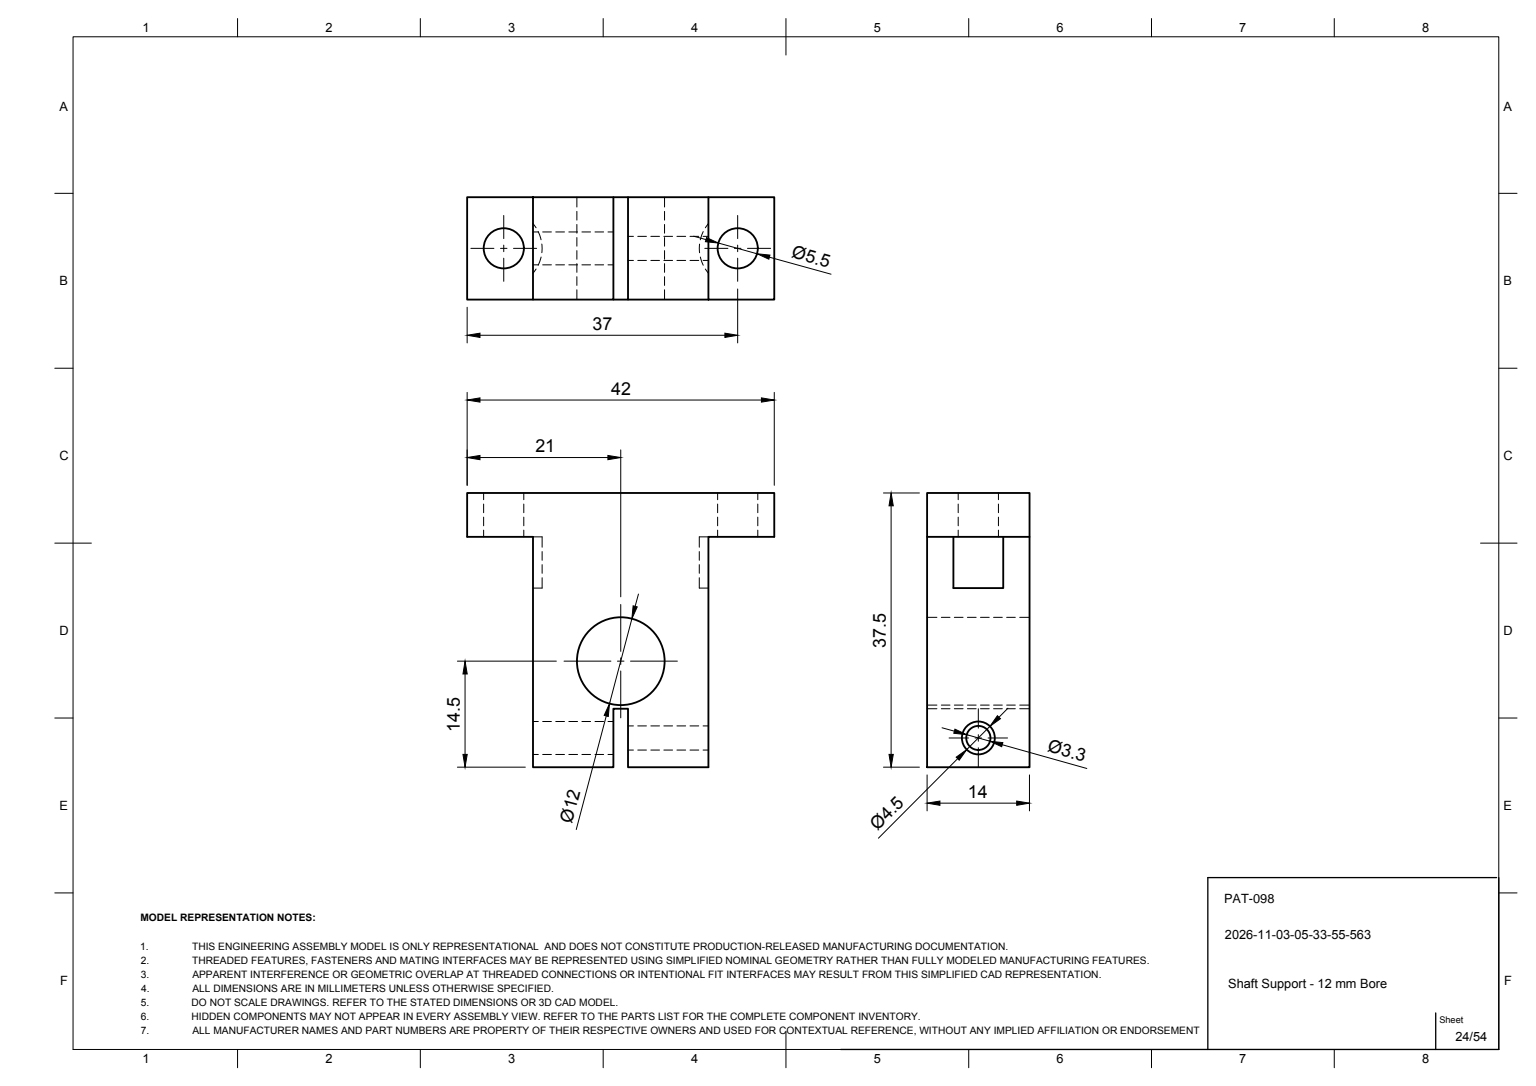
ISO-10303-21;
HEADER;
/* Generated by software containing ST-Developer
 * from STEP Tools, Inc. (www.steptools.com) 
 */

FILE_DESCRIPTION(
/* description */ ('Spring compression tester'),
/* implementation_level */ '2;1');

FILE_NAME(
/* name */ 'Shaft Support - 12 mm Bore.step',
/* time_stamp */ '2026-10-28T03:24:11-07:00',
/* author */ (''),
/* organization */ (''),
/* preprocessor_version */ 'ST-DEVELOPER v20.2',
/* originating_system */ 'Autodesk Translation Framework v15.17.0.0',
/* authorisation */ '');

FILE_SCHEMA (('AUTOMOTIVE_DESIGN { 1 0 10303 214 3 1 1 }'));
ENDSEC;

DATA;
#10=MECHANICAL_DESIGN_GEOMETRIC_PRESENTATION_REPRESENTATION('',(#1125),#43521);
#1005=SHAPE_REPRESENTATION_RELATIONSHIP('SRR','None',#43817,#1065);
#1065=ADVANCED_BREP_SHAPE_REPRESENTATION('',(#1200),#43477);
#1125=STYLED_ITEM('',(#44202),#1200);
#1200=MANIFOLD_SOLID_BREP('Body1',#18562);
#1439=FACE_BOUND('',#3801,.T.);
#1440=FACE_BOUND('',#3803,.T.);
#1441=FACE_BOUND('',#3805,.T.);
#1442=FACE_BOUND('',#3812,.T.);
#1443=FACE_BOUND('',#3815,.T.);
#1444=FACE_BOUND('',#3816,.T.);
#1445=FACE_BOUND('',#3819,.T.);
#1446=FACE_BOUND('',#3822,.T.);
#1447=FACE_BOUND('',#3825,.T.);
#1448=FACE_BOUND('',#3828,.T.);
#1861=PLANE('',#19931);
#1862=PLANE('',#19938);
#1863=PLANE('',#19939);
#1864=PLANE('',#19941);
#1865=PLANE('',#19943);
#1866=PLANE('',#19957);
#1867=PLANE('',#19958);
#1868=PLANE('',#19959);
#1869=PLANE('',#19960);
#1870=PLANE('',#19961);
#1871=PLANE('',#19962);
#1872=PLANE('',#19963);
#1873=PLANE('',#19964);
#1874=PLANE('',#19965);
#1875=PLANE('',#19966);
#1876=PLANE('',#19967);
#2557=FACE_OUTER_BOUND('',#3796,.T.);
#2558=FACE_OUTER_BOUND('',#3797,.T.);
#2559=FACE_OUTER_BOUND('',#3798,.T.);
#2560=FACE_OUTER_BOUND('',#3799,.T.);
#2561=FACE_OUTER_BOUND('',#3800,.T.);
#2562=FACE_OUTER_BOUND('',#3802,.T.);
#2563=FACE_OUTER_BOUND('',#3804,.T.);
#2564=FACE_OUTER_BOUND('',#3806,.T.);
#2565=FACE_OUTER_BOUND('',#3807,.T.);
#2566=FACE_OUTER_BOUND('',#3808,.T.);
#2567=FACE_OUTER_BOUND('',#3809,.T.);
#2568=FACE_OUTER_BOUND('',#3810,.T.);
#2569=FACE_OUTER_BOUND('',#3811,.T.);
#2570=FACE_OUTER_BOUND('',#3813,.T.);
#2571=FACE_OUTER_BOUND('',#3814,.T.);
#2572=FACE_OUTER_BOUND('',#3817,.T.);
#2573=FACE_OUTER_BOUND('',#3818,.T.);
#2574=FACE_OUTER_BOUND('',#3820,.T.);
#2575=FACE_OUTER_BOUND('',#3821,.T.);
#2576=FACE_OUTER_BOUND('',#3823,.T.);
#2577=FACE_OUTER_BOUND('',#3824,.T.);
#2578=FACE_OUTER_BOUND('',#3826,.T.);
#2579=FACE_OUTER_BOUND('',#3827,.T.);
#3796=EDGE_LOOP('',(#13935,#13936));
#3797=EDGE_LOOP('',(#13937,#13938,#13939,#13940));
#3798=EDGE_LOOP('',(#13941,#13942,#13943,#13944));
#3799=EDGE_LOOP('',(#13945,#13946));
#3800=EDGE_LOOP('',(#13947,#13948,#13949,#13950,#13951,#13952));
#3801=EDGE_LOOP('',(#13953));
#3802=EDGE_LOOP('',(#13954,#13955,#13956,#13957,#13958,#13959,#13960,#13961));
#3803=EDGE_LOOP('',(#13962));
#3804=EDGE_LOOP('',(#13963,#13964,#13965,#13966,#13967,#13968));
#3805=EDGE_LOOP('',(#13969));
#3806=EDGE_LOOP('',(#13970,#13971,#13972,#13973));
#3807=EDGE_LOOP('',(#13974,#13975,#13976,#13977));
#3808=EDGE_LOOP('',(#13978,#13979,#13980,#13981));
#3809=EDGE_LOOP('',(#13982,#13983,#13984,#13985));
#3810=EDGE_LOOP('',(#13986,#13987,#13988,#13989));
#3811=EDGE_LOOP('',(#13990,#13991,#13992,#13993,#13994,#13995,#13996,#13997,
#13998,#13999,#14000,#14001));
#3812=EDGE_LOOP('',(#14002));
#3813=EDGE_LOOP('',(#14003,#14004,#14005,#14006));
#3814=EDGE_LOOP('',(#14007,#14008,#14009,#14010));
#3815=EDGE_LOOP('',(#14011));
#3816=EDGE_LOOP('',(#14012));
#3817=EDGE_LOOP('',(#14013,#14014,#14015,#14016));
#3818=EDGE_LOOP('',(#14017,#14018,#14019,#14020,#14021,#14022,#14023,#14024));
#3819=EDGE_LOOP('',(#14025));
#3820=EDGE_LOOP('',(#14026,#14027,#14028,#14029));
#3821=EDGE_LOOP('',(#14030,#14031,#14032,#14033));
#3822=EDGE_LOOP('',(#14034));
#3823=EDGE_LOOP('',(#14035,#14036,#14037,#14038));
#3824=EDGE_LOOP('',(#14039,#14040,#14041,#14042));
#3825=EDGE_LOOP('',(#14043));
#3826=EDGE_LOOP('',(#14044,#14045,#14046,#14047));
#3827=EDGE_LOOP('',(#14048,#14049,#14050,#14051,#14052,#14053,#14054,#14055,
#14056,#14057,#14058,#14059));
#3828=EDGE_LOOP('',(#14060));
#5229=LINE('',#28297,#6661);
#5230=LINE('',#28301,#6662);
#5231=LINE('',#28304,#6663);
#5232=LINE('',#28308,#6664);
#5233=LINE('',#28312,#6665);
#5234=LINE('',#28315,#6666);
#5235=LINE('',#28318,#6667);
#5236=LINE('',#28320,#6668);
#5237=LINE('',#28322,#6669);
#5238=LINE('',#28324,#6670);
#5239=LINE('',#28325,#6671);
#5240=LINE('',#28330,#6672);
#5241=LINE('',#28332,#6673);
#5242=LINE('',#28333,#6674);
#5243=LINE('',#28339,#6675);
#5244=LINE('',#28341,#6676);
#5245=LINE('',#28342,#6677);
#5246=LINE('',#28344,#6678);
#5247=LINE('',#28345,#6679);
#5248=LINE('',#28352,#6680);
#5249=LINE('',#28356,#6681);
#5250=LINE('',#28361,#6682);
#5251=LINE('',#28365,#6683);
#5252=LINE('',#28370,#6684);
#5253=LINE('',#28374,#6685);
#5254=LINE('',#28376,#6686);
#5255=LINE('',#28377,#6687);
#5256=LINE('',#28379,#6688);
#5257=LINE('',#28381,#6689);
#5258=LINE('',#28383,#6690);
#5259=LINE('',#28385,#6691);
#5260=LINE('',#28387,#6692);
#5261=LINE('',#28388,#6693);
#5262=LINE('',#28391,#6694);
#5263=LINE('',#28392,#6695);
#5264=LINE('',#28395,#6696);
#5265=LINE('',#28396,#6697);
#5266=LINE('',#28398,#6698);
#5267=LINE('',#28401,#6699);
#5268=LINE('',#28402,#6700);
#5269=LINE('',#28405,#6701);
#5270=LINE('',#28406,#6702);
#5271=LINE('',#28409,#6703);
#5272=LINE('',#28410,#6704);
#5273=LINE('',#28413,#6705);
#5274=LINE('',#28414,#6706);
#5275=LINE('',#28417,#6707);
#5276=LINE('',#28418,#6708);
#5277=LINE('',#28420,#6709);
#6661=VECTOR('',#23115,1.);
#6662=VECTOR('',#23120,1.);
#6663=VECTOR('',#23123,1.);
#6664=VECTOR('',#23126,1.);
#6665=VECTOR('',#23129,1.);
#6666=VECTOR('',#23134,1.);
#6667=VECTOR('',#23137,1.);
#6668=VECTOR('',#23138,1.);
#6669=VECTOR('',#23139,1.);
#6670=VECTOR('',#23140,1.);
#6671=VECTOR('',#23141,1.);
#6672=VECTOR('',#23146,1.);
#6673=VECTOR('',#23147,1.);
#6674=VECTOR('',#23148,1.);
#6675=VECTOR('',#23153,1.);
#6676=VECTOR('',#23154,1.);
#6677=VECTOR('',#23155,1.);
#6678=VECTOR('',#23156,1.);
#6679=VECTOR('',#23157,1.);
#6680=VECTOR('',#23164,0.225);
#6681=VECTOR('',#23169,0.165);
#6682=VECTOR('',#23176,0.275);
#6683=VECTOR('',#23181,0.275);
#6684=VECTOR('',#23186,0.6);
#6685=VECTOR('',#23191,1.);
#6686=VECTOR('',#23192,1.);
#6687=VECTOR('',#23193,1.);
#6688=VECTOR('',#23194,1.);
#6689=VECTOR('',#23195,1.);
#6690=VECTOR('',#23196,1.);
#6691=VECTOR('',#23197,1.);
#6692=VECTOR('',#23198,1.);
#6693=VECTOR('',#23199,1.);
#6694=VECTOR('',#23202,1.);
#6695=VECTOR('',#23203,1.);
#6696=VECTOR('',#23206,1.);
#6697=VECTOR('',#23207,1.);
#6698=VECTOR('',#23210,1.);
#6699=VECTOR('',#23213,1.);
#6700=VECTOR('',#23214,1.);
#6701=VECTOR('',#23217,1.);
#6702=VECTOR('',#23218,1.);
#6703=VECTOR('',#23221,1.);
#6704=VECTOR('',#23222,1.);
#6705=VECTOR('',#23225,1.);
#6706=VECTOR('',#23226,1.);
#6707=VECTOR('',#23229,1.);
#6708=VECTOR('',#23230,1.);
#6709=VECTOR('',#23233,1.);
#7706=CIRCLE('',#19932,0.525);
#7707=CIRCLE('',#19934,0.525);
#7708=CIRCLE('',#19936,0.525);
#7709=CIRCLE('',#19937,0.525);
#7710=CIRCLE('',#19940,0.275);
#7711=CIRCLE('',#19942,0.165);
#7712=CIRCLE('',#19944,0.275);
#7713=CIRCLE('',#19946,0.225);
#7714=CIRCLE('',#19947,0.225);
#7715=CIRCLE('',#19949,0.165);
#7716=CIRCLE('',#19951,0.275);
#7717=CIRCLE('',#19953,0.275);
#7718=CIRCLE('',#19955,0.6);
#7719=CIRCLE('',#19956,0.6);
#8708=VERTEX_POINT('',#28295);
#8709=VERTEX_POINT('',#28296);
#8710=VERTEX_POINT('',#28300);
#8711=VERTEX_POINT('',#28302);
#8712=VERTEX_POINT('',#28306);
#8713=VERTEX_POINT('',#28307);
#8714=VERTEX_POINT('',#28309);
#8715=VERTEX_POINT('',#28311);
#8716=VERTEX_POINT('',#28317);
#8717=VERTEX_POINT('',#28319);
#8718=VERTEX_POINT('',#28321);
#8719=VERTEX_POINT('',#28323);
#8720=VERTEX_POINT('',#28326);
#8721=VERTEX_POINT('',#28329);
#8722=VERTEX_POINT('',#28331);
#8723=VERTEX_POINT('',#28334);
#8724=VERTEX_POINT('',#28337);
#8725=VERTEX_POINT('',#28338);
#8726=VERTEX_POINT('',#28340);
#8727=VERTEX_POINT('',#28343);
#8728=VERTEX_POINT('',#28346);
#8729=VERTEX_POINT('',#28349);
#8730=VERTEX_POINT('',#28351);
#8731=VERTEX_POINT('',#28355);
#8732=VERTEX_POINT('',#28359);
#8733=VERTEX_POINT('',#28363);
#8734=VERTEX_POINT('',#28367);
#8735=VERTEX_POINT('',#28369);
#8736=VERTEX_POINT('',#28373);
#8737=VERTEX_POINT('',#28375);
#8738=VERTEX_POINT('',#28378);
#8739=VERTEX_POINT('',#28380);
#8740=VERTEX_POINT('',#28382);
#8741=VERTEX_POINT('',#28384);
#8742=VERTEX_POINT('',#28386);
#8743=VERTEX_POINT('',#28390);
#8744=VERTEX_POINT('',#28394);
#8745=VERTEX_POINT('',#28400);
#8746=VERTEX_POINT('',#28404);
#8747=VERTEX_POINT('',#28408);
#8748=VERTEX_POINT('',#28412);
#8749=VERTEX_POINT('',#28416);
#10632=EDGE_CURVE('',#8708,#8709,#5229,.T.);
#10633=EDGE_CURVE('',#8709,#8708,#7706,.T.);
#10634=EDGE_CURVE('',#8710,#8708,#5230,.T.);
#10635=EDGE_CURVE('',#8711,#8710,#7707,.T.);
#10636=EDGE_CURVE('',#8709,#8711,#5231,.T.);
#10637=EDGE_CURVE('',#8712,#8713,#5232,.T.);
#10638=EDGE_CURVE('',#8712,#8714,#7708,.T.);
#10639=EDGE_CURVE('',#8715,#8714,#5233,.T.);
#10640=EDGE_CURVE('',#8713,#8715,#7709,.T.);
#10641=EDGE_CURVE('',#8714,#8712,#5234,.T.);
#10642=EDGE_CURVE('',#8710,#8716,#5235,.T.);
#10643=EDGE_CURVE('',#8717,#8716,#5236,.T.);
#10644=EDGE_CURVE('',#8717,#8718,#5237,.T.);
#10645=EDGE_CURVE('',#8719,#8718,#5238,.T.);
#10646=EDGE_CURVE('',#8719,#8711,#5239,.T.);
#10647=EDGE_CURVE('',#8720,#8720,#7710,.T.);
#10648=EDGE_CURVE('',#8721,#8719,#5240,.T.);
#10649=EDGE_CURVE('',#8721,#8722,#5241,.T.);
#10650=EDGE_CURVE('',#8716,#8722,#5242,.T.);
#10651=EDGE_CURVE('',#8723,#8723,#7711,.T.);
#10652=EDGE_CURVE('',#8724,#8725,#5243,.T.);
#10653=EDGE_CURVE('',#8726,#8725,#5244,.T.);
#10654=EDGE_CURVE('',#8713,#8726,#5245,.T.);
#10655=EDGE_CURVE('',#8727,#8715,#5246,.T.);
#10656=EDGE_CURVE('',#8724,#8727,#5247,.T.);
#10657=EDGE_CURVE('',#8728,#8728,#7712,.T.);
#10658=EDGE_CURVE('',#8729,#8729,#7713,.T.);
#10659=EDGE_CURVE('',#8729,#8730,#5248,.T.);
#10660=EDGE_CURVE('',#8730,#8730,#7714,.T.);
#10661=EDGE_CURVE('',#8723,#8731,#5249,.T.);
#10662=EDGE_CURVE('',#8731,#8731,#7715,.T.);
#10663=EDGE_CURVE('',#8732,#8732,#7716,.T.);
#10664=EDGE_CURVE('',#8732,#8720,#5250,.T.);
#10665=EDGE_CURVE('',#8733,#8733,#7717,.T.);
#10666=EDGE_CURVE('',#8733,#8728,#5251,.T.);
#10667=EDGE_CURVE('',#8734,#8734,#7718,.T.);
#10668=EDGE_CURVE('',#8734,#8735,#5252,.T.);
#10669=EDGE_CURVE('',#8735,#8735,#7719,.T.);
#10670=EDGE_CURVE('',#8718,#8736,#5253,.T.);
#10671=EDGE_CURVE('',#8736,#8737,#5254,.T.);
#10672=EDGE_CURVE('',#8737,#8724,#5255,.T.);
#10673=EDGE_CURVE('',#8727,#8738,#5256,.T.);
#10674=EDGE_CURVE('',#8738,#8739,#5257,.T.);
#10675=EDGE_CURVE('',#8739,#8740,#5258,.T.);
#10676=EDGE_CURVE('',#8740,#8741,#5259,.T.);
#10677=EDGE_CURVE('',#8741,#8742,#5260,.T.);
#10678=EDGE_CURVE('',#8742,#8721,#5261,.T.);
#10679=EDGE_CURVE('',#8743,#8717,#5262,.T.);
#10680=EDGE_CURVE('',#8736,#8743,#5263,.T.);
#10681=EDGE_CURVE('',#8744,#8743,#5264,.T.);
#10682=EDGE_CURVE('',#8737,#8744,#5265,.T.);
#10683=EDGE_CURVE('',#8725,#8744,#5266,.T.);
#10684=EDGE_CURVE('',#8745,#8726,#5267,.T.);
#10685=EDGE_CURVE('',#8738,#8745,#5268,.T.);
#10686=EDGE_CURVE('',#8746,#8745,#5269,.T.);
#10687=EDGE_CURVE('',#8739,#8746,#5270,.T.);
#10688=EDGE_CURVE('',#8747,#8746,#5271,.T.);
#10689=EDGE_CURVE('',#8740,#8747,#5272,.T.);
#10690=EDGE_CURVE('',#8748,#8747,#5273,.T.);
#10691=EDGE_CURVE('',#8741,#8748,#5274,.T.);
#10692=EDGE_CURVE('',#8749,#8748,#5275,.T.);
#10693=EDGE_CURVE('',#8742,#8749,#5276,.T.);
#10694=EDGE_CURVE('',#8722,#8749,#5277,.T.);
#13935=ORIENTED_EDGE('',*,*,#10632,.F.);
#13936=ORIENTED_EDGE('',*,*,#10633,.F.);
#13937=ORIENTED_EDGE('',*,*,#10634,.F.);
#13938=ORIENTED_EDGE('',*,*,#10635,.F.);
#13939=ORIENTED_EDGE('',*,*,#10636,.F.);
#13940=ORIENTED_EDGE('',*,*,#10633,.T.);
#13941=ORIENTED_EDGE('',*,*,#10637,.F.);
#13942=ORIENTED_EDGE('',*,*,#10638,.T.);
#13943=ORIENTED_EDGE('',*,*,#10639,.F.);
#13944=ORIENTED_EDGE('',*,*,#10640,.F.);
#13945=ORIENTED_EDGE('',*,*,#10641,.F.);
#13946=ORIENTED_EDGE('',*,*,#10638,.F.);
#13947=ORIENTED_EDGE('',*,*,#10642,.T.);
#13948=ORIENTED_EDGE('',*,*,#10643,.F.);
#13949=ORIENTED_EDGE('',*,*,#10644,.T.);
#13950=ORIENTED_EDGE('',*,*,#10645,.F.);
#13951=ORIENTED_EDGE('',*,*,#10646,.T.);
#13952=ORIENTED_EDGE('',*,*,#10635,.T.);
#13953=ORIENTED_EDGE('',*,*,#10647,.T.);
#13954=ORIENTED_EDGE('',*,*,#10634,.T.);
#13955=ORIENTED_EDGE('',*,*,#10632,.T.);
#13956=ORIENTED_EDGE('',*,*,#10636,.T.);
#13957=ORIENTED_EDGE('',*,*,#10646,.F.);
#13958=ORIENTED_EDGE('',*,*,#10648,.F.);
#13959=ORIENTED_EDGE('',*,*,#10649,.T.);
#13960=ORIENTED_EDGE('',*,*,#10650,.F.);
#13961=ORIENTED_EDGE('',*,*,#10642,.F.);
#13962=ORIENTED_EDGE('',*,*,#10651,.T.);
#13963=ORIENTED_EDGE('',*,*,#10652,.T.);
#13964=ORIENTED_EDGE('',*,*,#10653,.F.);
#13965=ORIENTED_EDGE('',*,*,#10654,.F.);
#13966=ORIENTED_EDGE('',*,*,#10640,.T.);
#13967=ORIENTED_EDGE('',*,*,#10655,.F.);
#13968=ORIENTED_EDGE('',*,*,#10656,.F.);
#13969=ORIENTED_EDGE('',*,*,#10657,.T.);
#13970=ORIENTED_EDGE('',*,*,#10658,.F.);
#13971=ORIENTED_EDGE('',*,*,#10659,.T.);
#13972=ORIENTED_EDGE('',*,*,#10660,.F.);
#13973=ORIENTED_EDGE('',*,*,#10659,.F.);
#13974=ORIENTED_EDGE('',*,*,#10651,.F.);
#13975=ORIENTED_EDGE('',*,*,#10661,.T.);
#13976=ORIENTED_EDGE('',*,*,#10662,.F.);
#13977=ORIENTED_EDGE('',*,*,#10661,.F.);
#13978=ORIENTED_EDGE('',*,*,#10663,.F.);
#13979=ORIENTED_EDGE('',*,*,#10664,.T.);
#13980=ORIENTED_EDGE('',*,*,#10647,.F.);
#13981=ORIENTED_EDGE('',*,*,#10664,.F.);
#13982=ORIENTED_EDGE('',*,*,#10665,.F.);
#13983=ORIENTED_EDGE('',*,*,#10666,.T.);
#13984=ORIENTED_EDGE('',*,*,#10657,.F.);
#13985=ORIENTED_EDGE('',*,*,#10666,.F.);
#13986=ORIENTED_EDGE('',*,*,#10667,.F.);
#13987=ORIENTED_EDGE('',*,*,#10668,.T.);
#13988=ORIENTED_EDGE('',*,*,#10669,.F.);
#13989=ORIENTED_EDGE('',*,*,#10668,.F.);
#13990=ORIENTED_EDGE('',*,*,#10645,.T.);
#13991=ORIENTED_EDGE('',*,*,#10670,.T.);
#13992=ORIENTED_EDGE('',*,*,#10671,.T.);
#13993=ORIENTED_EDGE('',*,*,#10672,.T.);
#13994=ORIENTED_EDGE('',*,*,#10656,.T.);
#13995=ORIENTED_EDGE('',*,*,#10673,.T.);
#13996=ORIENTED_EDGE('',*,*,#10674,.T.);
#13997=ORIENTED_EDGE('',*,*,#10675,.T.);
#13998=ORIENTED_EDGE('',*,*,#10676,.T.);
#13999=ORIENTED_EDGE('',*,*,#10677,.T.);
#14000=ORIENTED_EDGE('',*,*,#10678,.T.);
#14001=ORIENTED_EDGE('',*,*,#10648,.T.);
#14002=ORIENTED_EDGE('',*,*,#10667,.T.);
#14003=ORIENTED_EDGE('',*,*,#10644,.F.);
#14004=ORIENTED_EDGE('',*,*,#10679,.F.);
#14005=ORIENTED_EDGE('',*,*,#10680,.F.);
#14006=ORIENTED_EDGE('',*,*,#10670,.F.);
#14007=ORIENTED_EDGE('',*,*,#10680,.T.);
#14008=ORIENTED_EDGE('',*,*,#10681,.F.);
#14009=ORIENTED_EDGE('',*,*,#10682,.F.);
#14010=ORIENTED_EDGE('',*,*,#10671,.F.);
#14011=ORIENTED_EDGE('',*,*,#10663,.T.);
#14012=ORIENTED_EDGE('',*,*,#10665,.T.);
#14013=ORIENTED_EDGE('',*,*,#10682,.T.);
#14014=ORIENTED_EDGE('',*,*,#10683,.F.);
#14015=ORIENTED_EDGE('',*,*,#10652,.F.);
#14016=ORIENTED_EDGE('',*,*,#10672,.F.);
#14017=ORIENTED_EDGE('',*,*,#10637,.T.);
#14018=ORIENTED_EDGE('',*,*,#10654,.T.);
#14019=ORIENTED_EDGE('',*,*,#10684,.F.);
#14020=ORIENTED_EDGE('',*,*,#10685,.F.);
#14021=ORIENTED_EDGE('',*,*,#10673,.F.);
#14022=ORIENTED_EDGE('',*,*,#10655,.T.);
#14023=ORIENTED_EDGE('',*,*,#10639,.T.);
#14024=ORIENTED_EDGE('',*,*,#10641,.T.);
#14025=ORIENTED_EDGE('',*,*,#10660,.T.);
#14026=ORIENTED_EDGE('',*,*,#10685,.T.);
#14027=ORIENTED_EDGE('',*,*,#10686,.F.);
#14028=ORIENTED_EDGE('',*,*,#10687,.F.);
#14029=ORIENTED_EDGE('',*,*,#10674,.F.);
#14030=ORIENTED_EDGE('',*,*,#10687,.T.);
#14031=ORIENTED_EDGE('',*,*,#10688,.F.);
#14032=ORIENTED_EDGE('',*,*,#10689,.F.);
#14033=ORIENTED_EDGE('',*,*,#10675,.F.);
#14034=ORIENTED_EDGE('',*,*,#10658,.T.);
#14035=ORIENTED_EDGE('',*,*,#10689,.T.);
#14036=ORIENTED_EDGE('',*,*,#10690,.F.);
#14037=ORIENTED_EDGE('',*,*,#10691,.F.);
#14038=ORIENTED_EDGE('',*,*,#10676,.F.);
#14039=ORIENTED_EDGE('',*,*,#10691,.T.);
#14040=ORIENTED_EDGE('',*,*,#10692,.F.);
#14041=ORIENTED_EDGE('',*,*,#10693,.F.);
#14042=ORIENTED_EDGE('',*,*,#10677,.F.);
#14043=ORIENTED_EDGE('',*,*,#10662,.T.);
#14044=ORIENTED_EDGE('',*,*,#10693,.T.);
#14045=ORIENTED_EDGE('',*,*,#10694,.F.);
#14046=ORIENTED_EDGE('',*,*,#10649,.F.);
#14047=ORIENTED_EDGE('',*,*,#10678,.F.);
#14048=ORIENTED_EDGE('',*,*,#10643,.T.);
#14049=ORIENTED_EDGE('',*,*,#10650,.T.);
#14050=ORIENTED_EDGE('',*,*,#10694,.T.);
#14051=ORIENTED_EDGE('',*,*,#10692,.T.);
#14052=ORIENTED_EDGE('',*,*,#10690,.T.);
#14053=ORIENTED_EDGE('',*,*,#10688,.T.);
#14054=ORIENTED_EDGE('',*,*,#10686,.T.);
#14055=ORIENTED_EDGE('',*,*,#10684,.T.);
#14056=ORIENTED_EDGE('',*,*,#10653,.T.);
#14057=ORIENTED_EDGE('',*,*,#10683,.T.);
#14058=ORIENTED_EDGE('',*,*,#10681,.T.);
#14059=ORIENTED_EDGE('',*,*,#10679,.T.);
#14060=ORIENTED_EDGE('',*,*,#10669,.T.);
#17218=CYLINDRICAL_SURFACE('',#19933,0.525);
#17219=CYLINDRICAL_SURFACE('',#19935,0.525);
#17220=CYLINDRICAL_SURFACE('',#19945,0.225);
#17221=CYLINDRICAL_SURFACE('',#19948,0.165);
#17222=CYLINDRICAL_SURFACE('',#19950,0.275);
#17223=CYLINDRICAL_SURFACE('',#19952,0.275);
#17224=CYLINDRICAL_SURFACE('',#19954,0.6);
#17881=ADVANCED_FACE('',(#2557),#1861,.F.);
#17882=ADVANCED_FACE('',(#2558),#17218,.F.);
#17883=ADVANCED_FACE('',(#2559),#17219,.F.);
#17884=ADVANCED_FACE('',(#2560),#1862,.F.);
#17885=ADVANCED_FACE('',(#2561,#1439),#1863,.T.);
#17886=ADVANCED_FACE('',(#2562,#1440),#1864,.T.);
#17887=ADVANCED_FACE('',(#2563,#1441),#1865,.T.);
#17888=ADVANCED_FACE('',(#2564),#17220,.F.);
#17889=ADVANCED_FACE('',(#2565),#17221,.F.);
#17890=ADVANCED_FACE('',(#2566),#17222,.F.);
#17891=ADVANCED_FACE('',(#2567),#17223,.F.);
#17892=ADVANCED_FACE('',(#2568),#17224,.F.);
#17893=ADVANCED_FACE('',(#2569,#1442),#1866,.T.);
#17894=ADVANCED_FACE('',(#2570),#1867,.T.);
#17895=ADVANCED_FACE('',(#2571,#1443,#1444),#1868,.T.);
#17896=ADVANCED_FACE('',(#2572),#1869,.T.);
#17897=ADVANCED_FACE('',(#2573,#1445),#1870,.T.);
#17898=ADVANCED_FACE('',(#2574),#1871,.T.);
#17899=ADVANCED_FACE('',(#2575,#1446),#1872,.T.);
#17900=ADVANCED_FACE('',(#2576),#1873,.T.);
#17901=ADVANCED_FACE('',(#2577,#1447),#1874,.T.);
#17902=ADVANCED_FACE('',(#2578),#1875,.T.);
#17903=ADVANCED_FACE('',(#2579,#1448),#1876,.T.);
#18562=CLOSED_SHELL('',(#17881,#17882,#17883,#17884,#17885,#17886,#17887,
#17888,#17889,#17890,#17891,#17892,#17893,#17894,#17895,#17896,#17897,#17898,
#17899,#17900,#17901,#17902,#17903));
#19930=AXIS2_PLACEMENT_3D('',#28293,#23111,#23112);
#19931=AXIS2_PLACEMENT_3D('',#28294,#23113,#23114);
#19932=AXIS2_PLACEMENT_3D('',#28298,#23116,#23117);
#19933=AXIS2_PLACEMENT_3D('',#28299,#23118,#23119);
#19934=AXIS2_PLACEMENT_3D('',#28303,#23121,#23122);
#19935=AXIS2_PLACEMENT_3D('',#28305,#23124,#23125);
#19936=AXIS2_PLACEMENT_3D('',#28310,#23127,#23128);
#19937=AXIS2_PLACEMENT_3D('',#28313,#23130,#23131);
#19938=AXIS2_PLACEMENT_3D('',#28314,#23132,#23133);
#19939=AXIS2_PLACEMENT_3D('',#28316,#23135,#23136);
#19940=AXIS2_PLACEMENT_3D('',#28327,#23142,#23143);
#19941=AXIS2_PLACEMENT_3D('',#28328,#23144,#23145);
#19942=AXIS2_PLACEMENT_3D('',#28335,#23149,#23150);
#19943=AXIS2_PLACEMENT_3D('',#28336,#23151,#23152);
#19944=AXIS2_PLACEMENT_3D('',#28347,#23158,#23159);
#19945=AXIS2_PLACEMENT_3D('',#28348,#23160,#23161);
#19946=AXIS2_PLACEMENT_3D('',#28350,#23162,#23163);
#19947=AXIS2_PLACEMENT_3D('',#28353,#23165,#23166);
#19948=AXIS2_PLACEMENT_3D('',#28354,#23167,#23168);
#19949=AXIS2_PLACEMENT_3D('',#28357,#23170,#23171);
#19950=AXIS2_PLACEMENT_3D('',#28358,#23172,#23173);
#19951=AXIS2_PLACEMENT_3D('',#28360,#23174,#23175);
#19952=AXIS2_PLACEMENT_3D('',#28362,#23177,#23178);
#19953=AXIS2_PLACEMENT_3D('',#28364,#23179,#23180);
#19954=AXIS2_PLACEMENT_3D('',#28366,#23182,#23183);
#19955=AXIS2_PLACEMENT_3D('',#28368,#23184,#23185);
#19956=AXIS2_PLACEMENT_3D('',#28371,#23187,#23188);
#19957=AXIS2_PLACEMENT_3D('',#28372,#23189,#23190);
#19958=AXIS2_PLACEMENT_3D('',#28389,#23200,#23201);
#19959=AXIS2_PLACEMENT_3D('',#28393,#23204,#23205);
#19960=AXIS2_PLACEMENT_3D('',#28397,#23208,#23209);
#19961=AXIS2_PLACEMENT_3D('',#28399,#23211,#23212);
#19962=AXIS2_PLACEMENT_3D('',#28403,#23215,#23216);
#19963=AXIS2_PLACEMENT_3D('',#28407,#23219,#23220);
#19964=AXIS2_PLACEMENT_3D('',#28411,#23223,#23224);
#19965=AXIS2_PLACEMENT_3D('',#28415,#23227,#23228);
#19966=AXIS2_PLACEMENT_3D('',#28419,#23231,#23232);
#19967=AXIS2_PLACEMENT_3D('',#28421,#23234,#23235);
#23111=DIRECTION('axis',(0.,0.,1.));
#23112=DIRECTION('refdir',(1.,0.,0.));
#23113=DIRECTION('center_axis',(0.,0.,1.));
#23114=DIRECTION('ref_axis',(1.,0.,0.));
#23115=DIRECTION('',(0.,-1.,0.));
#23116=DIRECTION('center_axis',(0.,0.,1.));
#23117=DIRECTION('ref_axis',(1.,0.,0.));
#23118=DIRECTION('center_axis',(0.,0.,1.));
#23119=DIRECTION('ref_axis',(1.,0.,0.));
#23120=DIRECTION('',(0.,0.,1.));
#23121=DIRECTION('center_axis',(0.,0.,1.));
#23122=DIRECTION('ref_axis',(1.,0.,0.));
#23123=DIRECTION('',(0.,0.,-1.));
#23124=DIRECTION('center_axis',(0.,0.,1.));
#23125=DIRECTION('ref_axis',(-1.,1.22464679914735E-16,0.));
#23126=DIRECTION('',(0.,0.,-1.));
#23127=DIRECTION('center_axis',(0.,0.,1.));
#23128=DIRECTION('ref_axis',(1.,0.,0.));
#23129=DIRECTION('',(0.,0.,1.));
#23130=DIRECTION('center_axis',(0.,0.,1.));
#23131=DIRECTION('ref_axis',(1.,0.,0.));
#23132=DIRECTION('center_axis',(0.,0.,1.));
#23133=DIRECTION('ref_axis',(1.,0.,0.));
#23134=DIRECTION('',(0.,1.,0.));
#23135=DIRECTION('center_axis',(0.,0.,1.));
#23136=DIRECTION('ref_axis',(1.,0.,0.));
#23137=DIRECTION('',(0.,1.,0.));
#23138=DIRECTION('',(1.,0.,0.));
#23139=DIRECTION('',(0.,-1.,0.));
#23140=DIRECTION('',(-1.,0.,0.));
#23141=DIRECTION('',(0.,1.,0.));
#23142=DIRECTION('center_axis',(0.,0.,-1.));
#23143=DIRECTION('ref_axis',(1.,0.,0.));
#23144=DIRECTION('center_axis',(-1.,0.,0.));
#23145=DIRECTION('ref_axis',(0.,0.,1.));
#23146=DIRECTION('',(0.,0.,-1.));
#23147=DIRECTION('',(0.,1.,0.));
#23148=DIRECTION('',(0.,0.,1.));
#23149=DIRECTION('center_axis',(1.,0.,0.));
#23150=DIRECTION('ref_axis',(0.,0.,-1.));
#23151=DIRECTION('center_axis',(0.,0.,1.));
#23152=DIRECTION('ref_axis',(1.,0.,0.));
#23153=DIRECTION('',(0.,1.,0.));
#23154=DIRECTION('',(1.,0.,0.));
#23155=DIRECTION('',(0.,1.,0.));
#23156=DIRECTION('',(0.,1.,0.));
#23157=DIRECTION('',(-1.,0.,0.));
#23158=DIRECTION('center_axis',(0.,0.,-1.));
#23159=DIRECTION('ref_axis',(1.,0.,0.));
#23160=DIRECTION('center_axis',(1.,0.,0.));
#23161=DIRECTION('ref_axis',(0.,0.,-1.));
#23162=DIRECTION('center_axis',(1.,0.,0.));
#23163=DIRECTION('ref_axis',(0.,0.,-1.));
#23164=DIRECTION('',(1.,0.,0.));
#23165=DIRECTION('center_axis',(-1.,0.,0.));
#23166=DIRECTION('ref_axis',(0.,0.,-1.));
#23167=DIRECTION('center_axis',(1.,0.,0.));
#23168=DIRECTION('ref_axis',(0.,0.,-1.));
#23169=DIRECTION('',(1.,0.,0.));
#23170=DIRECTION('center_axis',(-1.,0.,0.));
#23171=DIRECTION('ref_axis',(0.,0.,-1.));
#23172=DIRECTION('center_axis',(0.,0.,1.));
#23173=DIRECTION('ref_axis',(1.,0.,0.));
#23174=DIRECTION('center_axis',(0.,0.,1.));
#23175=DIRECTION('ref_axis',(1.,0.,0.));
#23176=DIRECTION('',(0.,0.,1.));
#23177=DIRECTION('center_axis',(0.,0.,1.));
#23178=DIRECTION('ref_axis',(1.,0.,0.));
#23179=DIRECTION('center_axis',(0.,0.,1.));
#23180=DIRECTION('ref_axis',(1.,0.,0.));
#23181=DIRECTION('',(0.,0.,1.));
#23182=DIRECTION('center_axis',(0.,1.,0.));
#23183=DIRECTION('ref_axis',(1.,0.,0.));
#23184=DIRECTION('center_axis',(0.,1.,0.));
#23185=DIRECTION('ref_axis',(1.,0.,0.));
#23186=DIRECTION('',(0.,1.,0.));
#23187=DIRECTION('center_axis',(0.,-1.,0.));
#23188=DIRECTION('ref_axis',(1.,0.,0.));
#23189=DIRECTION('center_axis',(0.,-1.,0.));
#23190=DIRECTION('ref_axis',(0.,0.,-1.));
#23191=DIRECTION('',(0.,0.,-1.));
#23192=DIRECTION('',(1.,0.,0.));
#23193=DIRECTION('',(0.,0.,1.));
#23194=DIRECTION('',(0.,0.,1.));
#23195=DIRECTION('',(-1.,0.,0.));
#23196=DIRECTION('',(0.,0.,-1.));
#23197=DIRECTION('',(-1.,0.,0.));
#23198=DIRECTION('',(0.,0.,1.));
#23199=DIRECTION('',(-1.,0.,0.));
#23200=DIRECTION('center_axis',(-1.,0.,0.));
#23201=DIRECTION('ref_axis',(0.,0.,1.));
#23202=DIRECTION('',(0.,0.,1.));
#23203=DIRECTION('',(0.,1.,0.));
#23204=DIRECTION('center_axis',(0.,0.,-1.));
#23205=DIRECTION('ref_axis',(-1.,0.,0.));
#23206=DIRECTION('',(-1.,0.,0.));
#23207=DIRECTION('',(0.,1.,0.));
#23208=DIRECTION('center_axis',(1.,0.,0.));
#23209=DIRECTION('ref_axis',(0.,0.,-1.));
#23210=DIRECTION('',(0.,0.,-1.));
#23211=DIRECTION('center_axis',(1.,0.,0.));
#23212=DIRECTION('ref_axis',(0.,0.,-1.));
#23213=DIRECTION('',(0.,0.,-1.));
#23214=DIRECTION('',(0.,1.,0.));
#23215=DIRECTION('center_axis',(0.,0.,1.));
#23216=DIRECTION('ref_axis',(1.,0.,0.));
#23217=DIRECTION('',(1.,0.,0.));
#23218=DIRECTION('',(0.,1.,0.));
#23219=DIRECTION('center_axis',(-1.,0.,0.));
#23220=DIRECTION('ref_axis',(0.,0.,1.));
#23221=DIRECTION('',(0.,0.,1.));
#23222=DIRECTION('',(0.,1.,0.));
#23223=DIRECTION('center_axis',(0.,0.,1.));
#23224=DIRECTION('ref_axis',(1.,0.,0.));
#23225=DIRECTION('',(1.,0.,0.));
#23226=DIRECTION('',(0.,1.,0.));
#23227=DIRECTION('center_axis',(1.,0.,0.));
#23228=DIRECTION('ref_axis',(0.,0.,-1.));
#23229=DIRECTION('',(0.,0.,-1.));
#23230=DIRECTION('',(0.,1.,0.));
#23231=DIRECTION('center_axis',(0.,0.,1.));
#23232=DIRECTION('ref_axis',(1.,0.,0.));
#23233=DIRECTION('',(1.,0.,0.));
#23234=DIRECTION('center_axis',(0.,1.,0.));
#23235=DIRECTION('ref_axis',(0.,0.,1.));
#28293=CARTESIAN_POINT('',(0.,0.,0.));
#28294=CARTESIAN_POINT('Origin',(-1.6,0.,1.3));
#28295=CARTESIAN_POINT('',(-1.2,0.340036762718386,1.3));
#28296=CARTESIAN_POINT('',(-1.2,-0.340036762718386,1.3));
#28297=CARTESIAN_POINT('',(-1.2,0.,1.3));
#28298=CARTESIAN_POINT('Origin',(-1.6,0.,1.3));
#28299=CARTESIAN_POINT('Origin',(-1.6,0.,0.6));
#28300=CARTESIAN_POINT('',(-1.2,0.340036762718386,0.6));
#28301=CARTESIAN_POINT('',(-1.2,0.340036762718386,0.6));
#28302=CARTESIAN_POINT('',(-1.2,-0.340036762718386,0.6));
#28303=CARTESIAN_POINT('Origin',(-1.6,0.,0.6));
#28304=CARTESIAN_POINT('',(-1.2,-0.340036762718386,0.6));
#28305=CARTESIAN_POINT('Origin',(1.6,0.,0.6));
#28306=CARTESIAN_POINT('',(1.2,0.340036762718386,1.3));
#28307=CARTESIAN_POINT('',(1.2,0.340036762718386,0.6));
#28308=CARTESIAN_POINT('',(1.2,0.340036762718386,0.6));
#28309=CARTESIAN_POINT('',(1.2,-0.340036762718386,1.3));
#28310=CARTESIAN_POINT('Origin',(1.6,0.,1.3));
#28311=CARTESIAN_POINT('',(1.2,-0.340036762718386,0.6));
#28312=CARTESIAN_POINT('',(1.2,-0.340036762718386,0.6));
#28313=CARTESIAN_POINT('Origin',(1.6,0.,0.6));
#28314=CARTESIAN_POINT('Origin',(1.6,0.,1.3));
#28315=CARTESIAN_POINT('',(1.2,0.,1.3));
#28316=CARTESIAN_POINT('Origin',(-2.1,0.,0.6));
#28317=CARTESIAN_POINT('',(-1.2,0.7,0.6));
#28318=CARTESIAN_POINT('',(-1.2,0.,0.6));
#28319=CARTESIAN_POINT('',(-2.1,0.7,0.6));
#28320=CARTESIAN_POINT('',(-1.2,0.7,0.6));
#28321=CARTESIAN_POINT('',(-2.1,-0.7,0.6));
#28322=CARTESIAN_POINT('',(-2.1,0.,0.6));
#28323=CARTESIAN_POINT('',(-1.2,-0.7,0.6));
#28324=CARTESIAN_POINT('',(-1.2,-0.7,0.6));
#28325=CARTESIAN_POINT('',(-1.2,0.,0.6));
#28326=CARTESIAN_POINT('',(-1.875,3.36777869765522E-17,0.6));
#28327=CARTESIAN_POINT('Origin',(-1.6,0.,0.6));
#28328=CARTESIAN_POINT('Origin',(-1.2,0.,0.6));
#28329=CARTESIAN_POINT('',(-1.2,-0.7,3.75));
#28330=CARTESIAN_POINT('',(-1.2,-0.7,3.75));
#28331=CARTESIAN_POINT('',(-1.2,0.7,3.75));
#28332=CARTESIAN_POINT('',(-1.2,0.,3.75));
#28333=CARTESIAN_POINT('',(-1.2,0.7,3.75));
#28334=CARTESIAN_POINT('',(-1.2,-2.02066721859313E-17,3.515));
#28335=CARTESIAN_POINT('Origin',(-1.2,0.,3.35));
#28336=CARTESIAN_POINT('Origin',(1.2,0.,0.6));
#28337=CARTESIAN_POINT('',(2.1,-0.7,0.6));
#28338=CARTESIAN_POINT('',(2.1,0.7,0.6));
#28339=CARTESIAN_POINT('',(2.1,0.,0.6));
#28340=CARTESIAN_POINT('',(1.2,0.7,0.6));
#28341=CARTESIAN_POINT('',(2.1,0.7,0.6));
#28342=CARTESIAN_POINT('',(1.2,0.,0.6));
#28343=CARTESIAN_POINT('',(1.2,-0.7,0.6));
#28344=CARTESIAN_POINT('',(1.2,0.,0.6));
#28345=CARTESIAN_POINT('',(2.1,-0.7,0.6));
#28346=CARTESIAN_POINT('',(1.325,3.36777869765522E-17,0.6));
#28347=CARTESIAN_POINT('Origin',(1.6,0.,0.6));
#28348=CARTESIAN_POINT('Origin',(0.1,0.,3.35));
#28349=CARTESIAN_POINT('',(0.1,-2.75545529808155E-17,3.575));
#28350=CARTESIAN_POINT('Origin',(0.1,0.,3.35));
#28351=CARTESIAN_POINT('',(1.2,2.75545529808155E-17,3.575));
#28352=CARTESIAN_POINT('',(0.1,-2.75545529808155E-17,3.575));
#28353=CARTESIAN_POINT('Origin',(1.2,0.,3.35));
#28354=CARTESIAN_POINT('Origin',(0.,0.,3.35));
#28355=CARTESIAN_POINT('',(-0.1,2.02066721859313E-17,3.515));
#28356=CARTESIAN_POINT('',(0.,-2.02066721859313E-17,3.515));
#28357=CARTESIAN_POINT('Origin',(-0.1,0.,3.35));
#28358=CARTESIAN_POINT('Origin',(-1.6,0.,-0.05));
#28359=CARTESIAN_POINT('',(-1.875,-3.36777869765522E-17,0.));
#28360=CARTESIAN_POINT('Origin',(-1.6,0.,0.));
#28361=CARTESIAN_POINT('',(-1.875,-3.36777869765522E-17,-0.05));
#28362=CARTESIAN_POINT('Origin',(1.6,0.,-0.05));
#28363=CARTESIAN_POINT('',(1.325,-3.36777869765522E-17,0.));
#28364=CARTESIAN_POINT('Origin',(1.6,0.,0.));
#28365=CARTESIAN_POINT('',(1.325,-3.36777869765522E-17,-0.05));
#28366=CARTESIAN_POINT('Origin',(0.,0.,2.3));
#28367=CARTESIAN_POINT('',(-0.6,-0.7,2.3));
#28368=CARTESIAN_POINT('Origin',(0.,-0.7,2.3));
#28369=CARTESIAN_POINT('',(-0.6,0.7,2.3));
#28370=CARTESIAN_POINT('',(-0.6,0.,2.3));
#28371=CARTESIAN_POINT('Origin',(0.,0.7,2.3));
#28372=CARTESIAN_POINT('Origin',(0.,-0.7,1.875));
#28373=CARTESIAN_POINT('',(-2.1,-0.7,0.));
#28374=CARTESIAN_POINT('',(-2.1,-0.7,0.6));
#28375=CARTESIAN_POINT('',(2.1,-0.7,0.));
#28376=CARTESIAN_POINT('',(-2.1,-0.7,0.));
#28377=CARTESIAN_POINT('',(2.1,-0.7,0.));
#28378=CARTESIAN_POINT('',(1.2,-0.7,3.75));
#28379=CARTESIAN_POINT('',(1.2,-0.7,0.6));
#28380=CARTESIAN_POINT('',(0.1,-0.7,3.75));
#28381=CARTESIAN_POINT('',(1.2,-0.7,3.75));
#28382=CARTESIAN_POINT('',(0.1,-0.7,2.95));
#28383=CARTESIAN_POINT('',(0.1,-0.7,3.75));
#28384=CARTESIAN_POINT('',(-0.1,-0.7,2.95));
#28385=CARTESIAN_POINT('',(0.1,-0.7,2.95));
#28386=CARTESIAN_POINT('',(-0.1,-0.7,3.75));
#28387=CARTESIAN_POINT('',(-0.1,-0.7,2.95));
#28388=CARTESIAN_POINT('',(-0.1,-0.7,3.75));
#28389=CARTESIAN_POINT('Origin',(-2.1,0.,0.));
#28390=CARTESIAN_POINT('',(-2.1,0.7,0.));
#28391=CARTESIAN_POINT('',(-2.1,0.7,0.6));
#28392=CARTESIAN_POINT('',(-2.1,0.,0.));
#28393=CARTESIAN_POINT('Origin',(2.1,0.,0.));
#28394=CARTESIAN_POINT('',(2.1,0.7,0.));
#28395=CARTESIAN_POINT('',(-2.1,0.7,0.));
#28396=CARTESIAN_POINT('',(2.1,0.,0.));
#28397=CARTESIAN_POINT('Origin',(2.1,0.,0.6));
#28398=CARTESIAN_POINT('',(2.1,0.7,0.));
#28399=CARTESIAN_POINT('Origin',(1.2,0.,3.75));
#28400=CARTESIAN_POINT('',(1.2,0.7,3.75));
#28401=CARTESIAN_POINT('',(1.2,0.7,0.6));
#28402=CARTESIAN_POINT('',(1.2,0.,3.75));
#28403=CARTESIAN_POINT('Origin',(0.1,0.,3.75));
#28404=CARTESIAN_POINT('',(0.1,0.7,3.75));
#28405=CARTESIAN_POINT('',(1.2,0.7,3.75));
#28406=CARTESIAN_POINT('',(0.1,0.,3.75));
#28407=CARTESIAN_POINT('Origin',(0.1,0.,2.95));
#28408=CARTESIAN_POINT('',(0.1,0.7,2.95));
#28409=CARTESIAN_POINT('',(0.1,0.7,3.75));
#28410=CARTESIAN_POINT('',(0.1,0.,2.95));
#28411=CARTESIAN_POINT('Origin',(-0.1,0.,2.95));
#28412=CARTESIAN_POINT('',(-0.1,0.7,2.95));
#28413=CARTESIAN_POINT('',(0.1,0.7,2.95));
#28414=CARTESIAN_POINT('',(-0.1,0.,2.95));
#28415=CARTESIAN_POINT('Origin',(-0.1,0.,3.75));
#28416=CARTESIAN_POINT('',(-0.1,0.7,3.75));
#28417=CARTESIAN_POINT('',(-0.1,0.7,2.95));
#28418=CARTESIAN_POINT('',(-0.1,0.,3.75));
#28419=CARTESIAN_POINT('Origin',(-1.2,0.,3.75));
#28420=CARTESIAN_POINT('',(-0.1,0.7,3.75));
#28421=CARTESIAN_POINT('Origin',(0.,0.7,1.875));
#43409=UNCERTAINTY_MEASURE_WITH_UNIT(LENGTH_MEASURE(0.001),#43522,
'DISTANCE_ACCURACY_VALUE',
'Maximum model space distance between geometric entities at asserted c
onnectivities');
#43453=UNCERTAINTY_MEASURE_WITH_UNIT(LENGTH_MEASURE(0.001),#43522,
'DISTANCE_ACCURACY_VALUE',
'Maximum model space distance between geometric entities at asserted c
onnectivities');
#43477=(
GEOMETRIC_REPRESENTATION_CONTEXT(3)
GLOBAL_UNCERTAINTY_ASSIGNED_CONTEXT((#43409))
GLOBAL_UNIT_ASSIGNED_CONTEXT((#43522,#43524,#43525))
REPRESENTATION_CONTEXT('','3D')
);
#43521=(
GEOMETRIC_REPRESENTATION_CONTEXT(3)
GLOBAL_UNCERTAINTY_ASSIGNED_CONTEXT((#43453))
GLOBAL_UNIT_ASSIGNED_CONTEXT((#43522,#43524,#43525))
REPRESENTATION_CONTEXT('','3D')
);
#43522=(
LENGTH_UNIT()
NAMED_UNIT(*)
SI_UNIT(.CENTI.,.METRE.)
);
#43524=(
NAMED_UNIT(*)
PLANE_ANGLE_UNIT()
SI_UNIT($,.RADIAN.)
);
#43525=(
NAMED_UNIT(*)
SI_UNIT($,.STERADIAN.)
SOLID_ANGLE_UNIT()
);
#43549=SHAPE_DEFINITION_REPRESENTATION(#43616,#43817);
#43616=PRODUCT_DEFINITION_SHAPE('',$,#43885);
#43817=SHAPE_REPRESENTATION('',(#19930),#43477);
#43861=PRODUCT_DEFINITION_CONTEXT('part definition',#44064,'design');
#43885=PRODUCT_DEFINITION('Shaft Support - 12 mm Bore',
'Shaft Support - 12 mm Bore',#43952,#43861);
#43952=PRODUCT_DEFINITION_FORMATION('',$,#44089);
#44064=APPLICATION_CONTEXT(
'Core Data for Automotive Mechanical Design Process');
#44065=PRODUCT_CONTEXT('part definition',#44064,'mechanical');
#44089=PRODUCT('Shaft Support - 12 mm Bore',
'Shaft Support - 12 mm Bore','Shaft Support - 12 mm Bore',(#44065));
#44196=COLOUR_RGB('Grey',0.48,0.52,0.57);
#44197=FILL_AREA_STYLE_COLOUR('',#44196);
#44198=FILL_AREA_STYLE('',(#44197));
#44199=SURFACE_STYLE_FILL_AREA(#44198);
#44200=SURFACE_SIDE_STYLE('',(#44199));
#44201=SURFACE_STYLE_USAGE(.BOTH.,#44200);
#44202=PRESENTATION_STYLE_ASSIGNMENT((#44201));
ENDSEC;
END-ISO-10303-21;
